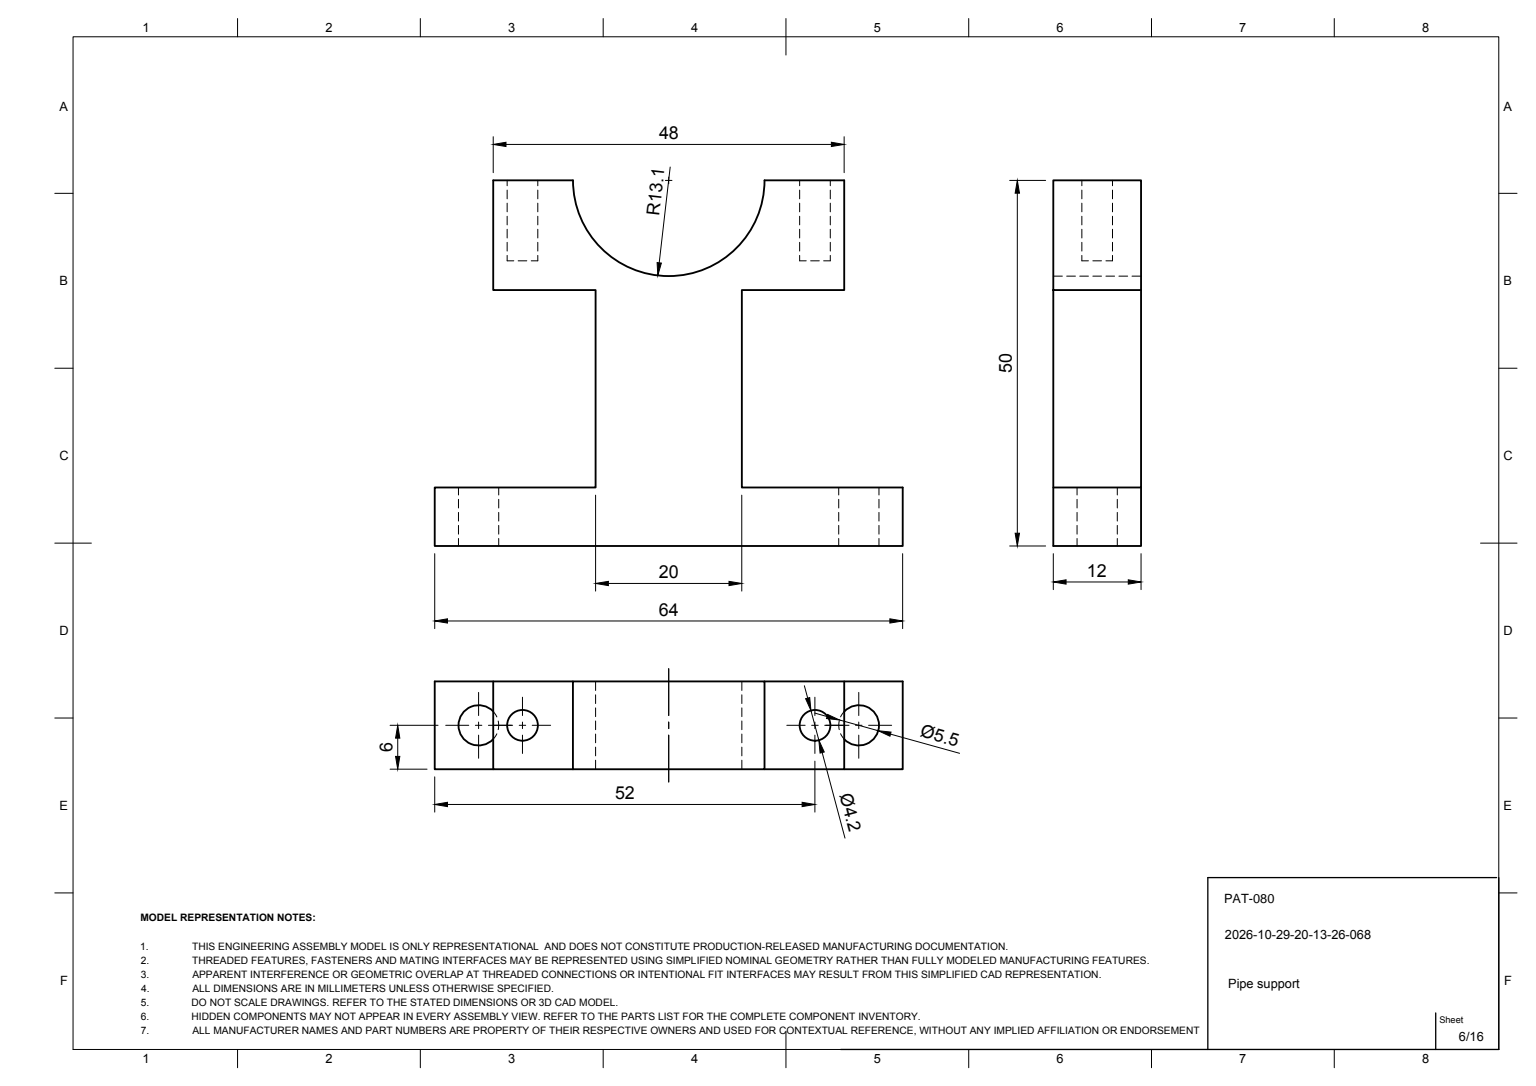
ISO-10303-21;
HEADER;
/* Generated by software containing ST-Developer
 * from STEP Tools, Inc. (www.steptools.com) 
 */

FILE_DESCRIPTION(
/* description */ ('PAT-080'),
/* implementation_level */ '2;1');

FILE_NAME(
/* name */ 'Pipe support.step',
/* time_stamp */ '2026-10-29T20:13:47-07:00',
/* author */ (''),
/* organization */ (''),
/* preprocessor_version */ 'ST-DEVELOPER v20.2',
/* originating_system */ 'Autodesk Translation Framework v15.17.0.0',
/* authorisation */ '');

FILE_SCHEMA (('AUTOMOTIVE_DESIGN { 1 0 10303 214 3 1 1 }'));
ENDSEC;

DATA;
#10=MECHANICAL_DESIGN_GEOMETRIC_PRESENTATION_REPRESENTATION('',(#249),#6878);
#211=SHAPE_REPRESENTATION_RELATIONSHIP('SRR','None',#6967,#230);
#230=ADVANCED_BREP_SHAPE_REPRESENTATION('',(#268),#6862);
#249=STYLED_ITEM('',(#7122),#268);
#268=MANIFOLD_SOLID_BREP('Body1',#3865);
#289=FACE_BOUND('',#765,.T.);
#290=FACE_BOUND('',#767,.T.);
#291=FACE_BOUND('',#769,.T.);
#292=FACE_BOUND('',#777,.T.);
#293=FACE_BOUND('',#780,.T.);
#294=FACE_BOUND('',#781,.T.);
#375=PLANE('',#4132);
#376=PLANE('',#4136);
#377=PLANE('',#4146);
#378=PLANE('',#4147);
#379=PLANE('',#4148);
#380=PLANE('',#4149);
#381=PLANE('',#4150);
#382=PLANE('',#4151);
#383=PLANE('',#4152);
#384=PLANE('',#4153);
#385=PLANE('',#4154);
#386=PLANE('',#4155);
#387=PLANE('',#4156);
#388=PLANE('',#4157);
#389=PLANE('',#4158);
#390=PLANE('',#4159);
#391=PLANE('',#4160);
#522=FACE_OUTER_BOUND('',#756,.T.);
#523=FACE_OUTER_BOUND('',#757,.T.);
#524=FACE_OUTER_BOUND('',#758,.T.);
#525=FACE_OUTER_BOUND('',#759,.T.);
#526=FACE_OUTER_BOUND('',#760,.T.);
#527=FACE_OUTER_BOUND('',#761,.T.);
#528=FACE_OUTER_BOUND('',#762,.T.);
#529=FACE_OUTER_BOUND('',#763,.T.);
#530=FACE_OUTER_BOUND('',#764,.T.);
#531=FACE_OUTER_BOUND('',#766,.T.);
#532=FACE_OUTER_BOUND('',#768,.T.);
#533=FACE_OUTER_BOUND('',#770,.T.);
#534=FACE_OUTER_BOUND('',#771,.T.);
#535=FACE_OUTER_BOUND('',#772,.T.);
#536=FACE_OUTER_BOUND('',#773,.T.);
#537=FACE_OUTER_BOUND('',#774,.T.);
#538=FACE_OUTER_BOUND('',#775,.T.);
#539=FACE_OUTER_BOUND('',#776,.T.);
#540=FACE_OUTER_BOUND('',#778,.T.);
#541=FACE_OUTER_BOUND('',#779,.T.);
#542=FACE_OUTER_BOUND('',#782,.T.);
#543=FACE_OUTER_BOUND('',#783,.T.);
#756=EDGE_LOOP('',(#2704,#2705,#2706,#2707));
#757=EDGE_LOOP('',(#2708));
#758=EDGE_LOOP('',(#2709,#2710,#2711,#2712));
#759=EDGE_LOOP('',(#2713));
#760=EDGE_LOOP('',(#2714,#2715,#2716,#2717));
#761=EDGE_LOOP('',(#2718,#2719,#2720,#2721));
#762=EDGE_LOOP('',(#2722,#2723,#2724,#2725));
#763=EDGE_LOOP('',(#2726,#2727,#2728,#2729,#2730,#2731,#2732,#2733,#2734,
#2735,#2736,#2737,#2738,#2739));
#764=EDGE_LOOP('',(#2740,#2741,#2742,#2743));
#765=EDGE_LOOP('',(#2744));
#766=EDGE_LOOP('',(#2745,#2746,#2747,#2748));
#767=EDGE_LOOP('',(#2749));
#768=EDGE_LOOP('',(#2750,#2751,#2752,#2753));
#769=EDGE_LOOP('',(#2754));
#770=EDGE_LOOP('',(#2755,#2756,#2757,#2758));
#771=EDGE_LOOP('',(#2759,#2760,#2761,#2762));
#772=EDGE_LOOP('',(#2763,#2764,#2765,#2766));
#773=EDGE_LOOP('',(#2767,#2768,#2769,#2770));
#774=EDGE_LOOP('',(#2771,#2772,#2773,#2774));
#775=EDGE_LOOP('',(#2775,#2776,#2777,#2778));
#776=EDGE_LOOP('',(#2779,#2780,#2781,#2782));
#777=EDGE_LOOP('',(#2783));
#778=EDGE_LOOP('',(#2784,#2785,#2786,#2787));
#779=EDGE_LOOP('',(#2788,#2789,#2790,#2791));
#780=EDGE_LOOP('',(#2792));
#781=EDGE_LOOP('',(#2793));
#782=EDGE_LOOP('',(#2794,#2795,#2796,#2797));
#783=EDGE_LOOP('',(#2798,#2799,#2800,#2801,#2802,#2803,#2804,#2805,#2806,
#2807,#2808,#2809,#2810,#2811));
#1068=LINE('',#5840,#1383);
#1069=LINE('',#5847,#1384);
#1070=LINE('',#5854,#1385);
#1071=LINE('',#5860,#1386);
#1072=LINE('',#5865,#1387);
#1073=LINE('',#5869,#1388);
#1074=LINE('',#5873,#1389);
#1075=LINE('',#5875,#1390);
#1076=LINE('',#5877,#1391);
#1077=LINE('',#5879,#1392);
#1078=LINE('',#5881,#1393);
#1079=LINE('',#5883,#1394);
#1080=LINE('',#5885,#1395);
#1081=LINE('',#5887,#1396);
#1082=LINE('',#5889,#1397);
#1083=LINE('',#5891,#1398);
#1084=LINE('',#5893,#1399);
#1085=LINE('',#5895,#1400);
#1086=LINE('',#5896,#1401);
#1087=LINE('',#5899,#1402);
#1088=LINE('',#5900,#1403);
#1089=LINE('',#5903,#1404);
#1090=LINE('',#5904,#1405);
#1091=LINE('',#5908,#1406);
#1092=LINE('',#5909,#1407);
#1093=LINE('',#5910,#1408);
#1094=LINE('',#5913,#1409);
#1095=LINE('',#5914,#1410);
#1096=LINE('',#5917,#1411);
#1097=LINE('',#5918,#1412);
#1098=LINE('',#5920,#1413);
#1099=LINE('',#5923,#1414);
#1100=LINE('',#5924,#1415);
#1101=LINE('',#5927,#1416);
#1102=LINE('',#5928,#1417);
#1103=LINE('',#5931,#1418);
#1104=LINE('',#5932,#1419);
#1105=LINE('',#5935,#1420);
#1106=LINE('',#5936,#1421);
#1107=LINE('',#5939,#1422);
#1108=LINE('',#5940,#1423);
#1109=LINE('',#5943,#1424);
#1110=LINE('',#5944,#1425);
#1111=LINE('',#5946,#1426);
#1383=VECTOR('',#4648,0.21);
#1384=VECTOR('',#4657,0.21);
#1385=VECTOR('',#4666,0.275);
#1386=VECTOR('',#4673,0.275);
#1387=VECTOR('',#4678,1.);
#1388=VECTOR('',#4681,1.);
#1389=VECTOR('',#4686,1.);
#1390=VECTOR('',#4687,1.);
#1391=VECTOR('',#4688,1.);
#1392=VECTOR('',#4689,1.);
#1393=VECTOR('',#4690,1.);
#1394=VECTOR('',#4691,1.);
#1395=VECTOR('',#4692,1.);
#1396=VECTOR('',#4693,1.);
#1397=VECTOR('',#4694,1.);
#1398=VECTOR('',#4695,1.);
#1399=VECTOR('',#4696,1.);
#1400=VECTOR('',#4697,1.);
#1401=VECTOR('',#4698,1.);
#1402=VECTOR('',#4701,1.);
#1403=VECTOR('',#4702,1.);
#1404=VECTOR('',#4705,1.);
#1405=VECTOR('',#4706,1.);
#1406=VECTOR('',#4709,1.);
#1407=VECTOR('',#4710,1.);
#1408=VECTOR('',#4711,1.);
#1409=VECTOR('',#4714,1.);
#1410=VECTOR('',#4715,1.);
#1411=VECTOR('',#4718,1.);
#1412=VECTOR('',#4719,1.);
#1413=VECTOR('',#4722,1.);
#1414=VECTOR('',#4725,1.);
#1415=VECTOR('',#4726,1.);
#1416=VECTOR('',#4729,1.);
#1417=VECTOR('',#4730,1.);
#1418=VECTOR('',#4733,1.);
#1419=VECTOR('',#4734,1.);
#1420=VECTOR('',#4737,1.);
#1421=VECTOR('',#4738,1.);
#1422=VECTOR('',#4741,1.);
#1423=VECTOR('',#4742,1.);
#1424=VECTOR('',#4745,1.);
#1425=VECTOR('',#4746,1.);
#1426=VECTOR('',#4749,1.);
#1666=CIRCLE('',#4130,0.21);
#1667=CIRCLE('',#4131,0.21);
#1668=CIRCLE('',#4134,0.21);
#1669=CIRCLE('',#4135,0.21);
#1670=CIRCLE('',#4138,0.275);
#1671=CIRCLE('',#4139,0.275);
#1672=CIRCLE('',#4141,0.275);
#1673=CIRCLE('',#4142,0.275);
#1674=CIRCLE('',#4144,1.31);
#1675=CIRCLE('',#4145,1.31);
#1842=VERTEX_POINT('',#5837);
#1843=VERTEX_POINT('',#5839);
#1844=VERTEX_POINT('',#5844);
#1845=VERTEX_POINT('',#5846);
#1846=VERTEX_POINT('',#5851);
#1847=VERTEX_POINT('',#5853);
#1848=VERTEX_POINT('',#5857);
#1849=VERTEX_POINT('',#5859);
#1850=VERTEX_POINT('',#5863);
#1851=VERTEX_POINT('',#5864);
#1852=VERTEX_POINT('',#5866);
#1853=VERTEX_POINT('',#5868);
#1854=VERTEX_POINT('',#5872);
#1855=VERTEX_POINT('',#5874);
#1856=VERTEX_POINT('',#5876);
#1857=VERTEX_POINT('',#5878);
#1858=VERTEX_POINT('',#5880);
#1859=VERTEX_POINT('',#5882);
#1860=VERTEX_POINT('',#5884);
#1861=VERTEX_POINT('',#5886);
#1862=VERTEX_POINT('',#5888);
#1863=VERTEX_POINT('',#5890);
#1864=VERTEX_POINT('',#5892);
#1865=VERTEX_POINT('',#5894);
#1866=VERTEX_POINT('',#5898);
#1867=VERTEX_POINT('',#5902);
#1868=VERTEX_POINT('',#5906);
#1869=VERTEX_POINT('',#5907);
#1870=VERTEX_POINT('',#5912);
#1871=VERTEX_POINT('',#5916);
#1872=VERTEX_POINT('',#5922);
#1873=VERTEX_POINT('',#5926);
#1874=VERTEX_POINT('',#5930);
#1875=VERTEX_POINT('',#5934);
#1876=VERTEX_POINT('',#5938);
#1877=VERTEX_POINT('',#5942);
#2175=EDGE_CURVE('',#1842,#1842,#1666,.T.);
#2176=EDGE_CURVE('',#1842,#1843,#1068,.T.);
#2177=EDGE_CURVE('',#1843,#1843,#1667,.T.);
#2178=EDGE_CURVE('',#1844,#1844,#1668,.T.);
#2179=EDGE_CURVE('',#1844,#1845,#1069,.T.);
#2180=EDGE_CURVE('',#1845,#1845,#1669,.T.);
#2181=EDGE_CURVE('',#1846,#1846,#1670,.T.);
#2182=EDGE_CURVE('',#1846,#1847,#1070,.T.);
#2183=EDGE_CURVE('',#1847,#1847,#1671,.T.);
#2184=EDGE_CURVE('',#1848,#1848,#1672,.T.);
#2185=EDGE_CURVE('',#1848,#1849,#1071,.T.);
#2186=EDGE_CURVE('',#1849,#1849,#1673,.T.);
#2187=EDGE_CURVE('',#1850,#1851,#1072,.T.);
#2188=EDGE_CURVE('',#1852,#1850,#1674,.T.);
#2189=EDGE_CURVE('',#1853,#1852,#1073,.T.);
#2190=EDGE_CURVE('',#1851,#1853,#1675,.T.);
#2191=EDGE_CURVE('',#1850,#1854,#1074,.T.);
#2192=EDGE_CURVE('',#1854,#1855,#1075,.T.);
#2193=EDGE_CURVE('',#1855,#1856,#1076,.T.);
#2194=EDGE_CURVE('',#1856,#1857,#1077,.T.);
#2195=EDGE_CURVE('',#1857,#1858,#1078,.T.);
#2196=EDGE_CURVE('',#1858,#1859,#1079,.T.);
#2197=EDGE_CURVE('',#1859,#1860,#1080,.T.);
#2198=EDGE_CURVE('',#1860,#1861,#1081,.T.);
#2199=EDGE_CURVE('',#1861,#1862,#1082,.T.);
#2200=EDGE_CURVE('',#1862,#1863,#1083,.T.);
#2201=EDGE_CURVE('',#1863,#1864,#1084,.T.);
#2202=EDGE_CURVE('',#1864,#1865,#1085,.T.);
#2203=EDGE_CURVE('',#1865,#1852,#1086,.T.);
#2204=EDGE_CURVE('',#1851,#1866,#1087,.T.);
#2205=EDGE_CURVE('',#1866,#1854,#1088,.T.);
#2206=EDGE_CURVE('',#1867,#1865,#1089,.T.);
#2207=EDGE_CURVE('',#1867,#1853,#1090,.T.);
#2208=EDGE_CURVE('',#1868,#1869,#1091,.T.);
#2209=EDGE_CURVE('',#1869,#1858,#1092,.T.);
#2210=EDGE_CURVE('',#1868,#1857,#1093,.T.);
#2211=EDGE_CURVE('',#1870,#1868,#1094,.T.);
#2212=EDGE_CURVE('',#1870,#1856,#1095,.T.);
#2213=EDGE_CURVE('',#1871,#1870,#1096,.T.);
#2214=EDGE_CURVE('',#1871,#1855,#1097,.T.);
#2215=EDGE_CURVE('',#1866,#1871,#1098,.T.);
#2216=EDGE_CURVE('',#1872,#1867,#1099,.T.);
#2217=EDGE_CURVE('',#1872,#1864,#1100,.T.);
#2218=EDGE_CURVE('',#1873,#1872,#1101,.T.);
#2219=EDGE_CURVE('',#1873,#1863,#1102,.T.);
#2220=EDGE_CURVE('',#1874,#1873,#1103,.T.);
#2221=EDGE_CURVE('',#1874,#1862,#1104,.T.);
#2222=EDGE_CURVE('',#1875,#1874,#1105,.T.);
#2223=EDGE_CURVE('',#1875,#1861,#1106,.T.);
#2224=EDGE_CURVE('',#1876,#1875,#1107,.T.);
#2225=EDGE_CURVE('',#1876,#1860,#1108,.T.);
#2226=EDGE_CURVE('',#1877,#1876,#1109,.T.);
#2227=EDGE_CURVE('',#1877,#1859,#1110,.T.);
#2228=EDGE_CURVE('',#1869,#1877,#1111,.T.);
#2704=ORIENTED_EDGE('',*,*,#2175,.F.);
#2705=ORIENTED_EDGE('',*,*,#2176,.T.);
#2706=ORIENTED_EDGE('',*,*,#2177,.F.);
#2707=ORIENTED_EDGE('',*,*,#2176,.F.);
#2708=ORIENTED_EDGE('',*,*,#2175,.T.);
#2709=ORIENTED_EDGE('',*,*,#2178,.F.);
#2710=ORIENTED_EDGE('',*,*,#2179,.T.);
#2711=ORIENTED_EDGE('',*,*,#2180,.F.);
#2712=ORIENTED_EDGE('',*,*,#2179,.F.);
#2713=ORIENTED_EDGE('',*,*,#2178,.T.);
#2714=ORIENTED_EDGE('',*,*,#2181,.F.);
#2715=ORIENTED_EDGE('',*,*,#2182,.T.);
#2716=ORIENTED_EDGE('',*,*,#2183,.F.);
#2717=ORIENTED_EDGE('',*,*,#2182,.F.);
#2718=ORIENTED_EDGE('',*,*,#2184,.F.);
#2719=ORIENTED_EDGE('',*,*,#2185,.T.);
#2720=ORIENTED_EDGE('',*,*,#2186,.F.);
#2721=ORIENTED_EDGE('',*,*,#2185,.F.);
#2722=ORIENTED_EDGE('',*,*,#2187,.F.);
#2723=ORIENTED_EDGE('',*,*,#2188,.F.);
#2724=ORIENTED_EDGE('',*,*,#2189,.F.);
#2725=ORIENTED_EDGE('',*,*,#2190,.F.);
#2726=ORIENTED_EDGE('',*,*,#2188,.T.);
#2727=ORIENTED_EDGE('',*,*,#2191,.T.);
#2728=ORIENTED_EDGE('',*,*,#2192,.T.);
#2729=ORIENTED_EDGE('',*,*,#2193,.T.);
#2730=ORIENTED_EDGE('',*,*,#2194,.T.);
#2731=ORIENTED_EDGE('',*,*,#2195,.T.);
#2732=ORIENTED_EDGE('',*,*,#2196,.T.);
#2733=ORIENTED_EDGE('',*,*,#2197,.T.);
#2734=ORIENTED_EDGE('',*,*,#2198,.T.);
#2735=ORIENTED_EDGE('',*,*,#2199,.T.);
#2736=ORIENTED_EDGE('',*,*,#2200,.T.);
#2737=ORIENTED_EDGE('',*,*,#2201,.T.);
#2738=ORIENTED_EDGE('',*,*,#2202,.T.);
#2739=ORIENTED_EDGE('',*,*,#2203,.T.);
#2740=ORIENTED_EDGE('',*,*,#2187,.T.);
#2741=ORIENTED_EDGE('',*,*,#2204,.T.);
#2742=ORIENTED_EDGE('',*,*,#2205,.T.);
#2743=ORIENTED_EDGE('',*,*,#2191,.F.);
#2744=ORIENTED_EDGE('',*,*,#2177,.T.);
#2745=ORIENTED_EDGE('',*,*,#2189,.T.);
#2746=ORIENTED_EDGE('',*,*,#2203,.F.);
#2747=ORIENTED_EDGE('',*,*,#2206,.F.);
#2748=ORIENTED_EDGE('',*,*,#2207,.T.);
#2749=ORIENTED_EDGE('',*,*,#2180,.T.);
#2750=ORIENTED_EDGE('',*,*,#2208,.T.);
#2751=ORIENTED_EDGE('',*,*,#2209,.T.);
#2752=ORIENTED_EDGE('',*,*,#2195,.F.);
#2753=ORIENTED_EDGE('',*,*,#2210,.F.);
#2754=ORIENTED_EDGE('',*,*,#2183,.T.);
#2755=ORIENTED_EDGE('',*,*,#2211,.T.);
#2756=ORIENTED_EDGE('',*,*,#2210,.T.);
#2757=ORIENTED_EDGE('',*,*,#2194,.F.);
#2758=ORIENTED_EDGE('',*,*,#2212,.F.);
#2759=ORIENTED_EDGE('',*,*,#2213,.T.);
#2760=ORIENTED_EDGE('',*,*,#2212,.T.);
#2761=ORIENTED_EDGE('',*,*,#2193,.F.);
#2762=ORIENTED_EDGE('',*,*,#2214,.F.);
#2763=ORIENTED_EDGE('',*,*,#2215,.T.);
#2764=ORIENTED_EDGE('',*,*,#2214,.T.);
#2765=ORIENTED_EDGE('',*,*,#2192,.F.);
#2766=ORIENTED_EDGE('',*,*,#2205,.F.);
#2767=ORIENTED_EDGE('',*,*,#2216,.T.);
#2768=ORIENTED_EDGE('',*,*,#2206,.T.);
#2769=ORIENTED_EDGE('',*,*,#2202,.F.);
#2770=ORIENTED_EDGE('',*,*,#2217,.F.);
#2771=ORIENTED_EDGE('',*,*,#2218,.T.);
#2772=ORIENTED_EDGE('',*,*,#2217,.T.);
#2773=ORIENTED_EDGE('',*,*,#2201,.F.);
#2774=ORIENTED_EDGE('',*,*,#2219,.F.);
#2775=ORIENTED_EDGE('',*,*,#2220,.T.);
#2776=ORIENTED_EDGE('',*,*,#2219,.T.);
#2777=ORIENTED_EDGE('',*,*,#2200,.F.);
#2778=ORIENTED_EDGE('',*,*,#2221,.F.);
#2779=ORIENTED_EDGE('',*,*,#2222,.T.);
#2780=ORIENTED_EDGE('',*,*,#2221,.T.);
#2781=ORIENTED_EDGE('',*,*,#2199,.F.);
#2782=ORIENTED_EDGE('',*,*,#2223,.F.);
#2783=ORIENTED_EDGE('',*,*,#2186,.T.);
#2784=ORIENTED_EDGE('',*,*,#2224,.T.);
#2785=ORIENTED_EDGE('',*,*,#2223,.T.);
#2786=ORIENTED_EDGE('',*,*,#2198,.F.);
#2787=ORIENTED_EDGE('',*,*,#2225,.F.);
#2788=ORIENTED_EDGE('',*,*,#2226,.T.);
#2789=ORIENTED_EDGE('',*,*,#2225,.T.);
#2790=ORIENTED_EDGE('',*,*,#2197,.F.);
#2791=ORIENTED_EDGE('',*,*,#2227,.F.);
#2792=ORIENTED_EDGE('',*,*,#2181,.T.);
#2793=ORIENTED_EDGE('',*,*,#2184,.T.);
#2794=ORIENTED_EDGE('',*,*,#2228,.T.);
#2795=ORIENTED_EDGE('',*,*,#2227,.T.);
#2796=ORIENTED_EDGE('',*,*,#2196,.F.);
#2797=ORIENTED_EDGE('',*,*,#2209,.F.);
#2798=ORIENTED_EDGE('',*,*,#2190,.T.);
#2799=ORIENTED_EDGE('',*,*,#2207,.F.);
#2800=ORIENTED_EDGE('',*,*,#2216,.F.);
#2801=ORIENTED_EDGE('',*,*,#2218,.F.);
#2802=ORIENTED_EDGE('',*,*,#2220,.F.);
#2803=ORIENTED_EDGE('',*,*,#2222,.F.);
#2804=ORIENTED_EDGE('',*,*,#2224,.F.);
#2805=ORIENTED_EDGE('',*,*,#2226,.F.);
#2806=ORIENTED_EDGE('',*,*,#2228,.F.);
#2807=ORIENTED_EDGE('',*,*,#2208,.F.);
#2808=ORIENTED_EDGE('',*,*,#2211,.F.);
#2809=ORIENTED_EDGE('',*,*,#2213,.F.);
#2810=ORIENTED_EDGE('',*,*,#2215,.F.);
#2811=ORIENTED_EDGE('',*,*,#2204,.F.);
#3574=CYLINDRICAL_SURFACE('',#4129,0.21);
#3575=CYLINDRICAL_SURFACE('',#4133,0.21);
#3576=CYLINDRICAL_SURFACE('',#4137,0.275);
#3577=CYLINDRICAL_SURFACE('',#4140,0.275);
#3578=CYLINDRICAL_SURFACE('',#4143,1.31);
#3658=ADVANCED_FACE('',(#522),#3574,.F.);
#3659=ADVANCED_FACE('',(#523),#375,.T.);
#3660=ADVANCED_FACE('',(#524),#3575,.F.);
#3661=ADVANCED_FACE('',(#525),#376,.T.);
#3662=ADVANCED_FACE('',(#526),#3576,.F.);
#3663=ADVANCED_FACE('',(#527),#3577,.F.);
#3664=ADVANCED_FACE('',(#528),#3578,.F.);
#3665=ADVANCED_FACE('',(#529),#377,.T.);
#3666=ADVANCED_FACE('',(#530,#289),#378,.T.);
#3667=ADVANCED_FACE('',(#531,#290),#379,.T.);
#3668=ADVANCED_FACE('',(#532,#291),#380,.T.);
#3669=ADVANCED_FACE('',(#533),#381,.T.);
#3670=ADVANCED_FACE('',(#534),#382,.T.);
#3671=ADVANCED_FACE('',(#535),#383,.T.);
#3672=ADVANCED_FACE('',(#536),#384,.T.);
#3673=ADVANCED_FACE('',(#537),#385,.T.);
#3674=ADVANCED_FACE('',(#538),#386,.T.);
#3675=ADVANCED_FACE('',(#539,#292),#387,.T.);
#3676=ADVANCED_FACE('',(#540),#388,.T.);
#3677=ADVANCED_FACE('',(#541,#293,#294),#389,.T.);
#3678=ADVANCED_FACE('',(#542),#390,.T.);
#3679=ADVANCED_FACE('',(#543),#391,.F.);
#3865=CLOSED_SHELL('',(#3658,#3659,#3660,#3661,#3662,#3663,#3664,#3665,
#3666,#3667,#3668,#3669,#3670,#3671,#3672,#3673,#3674,#3675,#3676,#3677,
#3678,#3679));
#4128=AXIS2_PLACEMENT_3D('',#5835,#4642,#4643);
#4129=AXIS2_PLACEMENT_3D('',#5836,#4644,#4645);
#4130=AXIS2_PLACEMENT_3D('',#5838,#4646,#4647);
#4131=AXIS2_PLACEMENT_3D('',#5841,#4649,#4650);
#4132=AXIS2_PLACEMENT_3D('',#5842,#4651,#4652);
#4133=AXIS2_PLACEMENT_3D('',#5843,#4653,#4654);
#4134=AXIS2_PLACEMENT_3D('',#5845,#4655,#4656);
#4135=AXIS2_PLACEMENT_3D('',#5848,#4658,#4659);
#4136=AXIS2_PLACEMENT_3D('',#5849,#4660,#4661);
#4137=AXIS2_PLACEMENT_3D('',#5850,#4662,#4663);
#4138=AXIS2_PLACEMENT_3D('',#5852,#4664,#4665);
#4139=AXIS2_PLACEMENT_3D('',#5855,#4667,#4668);
#4140=AXIS2_PLACEMENT_3D('',#5856,#4669,#4670);
#4141=AXIS2_PLACEMENT_3D('',#5858,#4671,#4672);
#4142=AXIS2_PLACEMENT_3D('',#5861,#4674,#4675);
#4143=AXIS2_PLACEMENT_3D('',#5862,#4676,#4677);
#4144=AXIS2_PLACEMENT_3D('',#5867,#4679,#4680);
#4145=AXIS2_PLACEMENT_3D('',#5870,#4682,#4683);
#4146=AXIS2_PLACEMENT_3D('',#5871,#4684,#4685);
#4147=AXIS2_PLACEMENT_3D('',#5897,#4699,#4700);
#4148=AXIS2_PLACEMENT_3D('',#5901,#4703,#4704);
#4149=AXIS2_PLACEMENT_3D('',#5905,#4707,#4708);
#4150=AXIS2_PLACEMENT_3D('',#5911,#4712,#4713);
#4151=AXIS2_PLACEMENT_3D('',#5915,#4716,#4717);
#4152=AXIS2_PLACEMENT_3D('',#5919,#4720,#4721);
#4153=AXIS2_PLACEMENT_3D('',#5921,#4723,#4724);
#4154=AXIS2_PLACEMENT_3D('',#5925,#4727,#4728);
#4155=AXIS2_PLACEMENT_3D('',#5929,#4731,#4732);
#4156=AXIS2_PLACEMENT_3D('',#5933,#4735,#4736);
#4157=AXIS2_PLACEMENT_3D('',#5937,#4739,#4740);
#4158=AXIS2_PLACEMENT_3D('',#5941,#4743,#4744);
#4159=AXIS2_PLACEMENT_3D('',#5945,#4747,#4748);
#4160=AXIS2_PLACEMENT_3D('',#5947,#4750,#4751);
#4642=DIRECTION('axis',(0.,0.,1.));
#4643=DIRECTION('refdir',(1.,0.,0.));
#4644=DIRECTION('center_axis',(0.,0.,1.));
#4645=DIRECTION('ref_axis',(1.,0.,0.));
#4646=DIRECTION('center_axis',(0.,0.,1.));
#4647=DIRECTION('ref_axis',(1.,0.,0.));
#4648=DIRECTION('',(0.,0.,1.));
#4649=DIRECTION('center_axis',(0.,0.,-1.));
#4650=DIRECTION('ref_axis',(1.,0.,0.));
#4651=DIRECTION('center_axis',(0.,0.,1.));
#4652=DIRECTION('ref_axis',(1.,0.,0.));
#4653=DIRECTION('center_axis',(0.,0.,1.));
#4654=DIRECTION('ref_axis',(1.,0.,0.));
#4655=DIRECTION('center_axis',(0.,0.,1.));
#4656=DIRECTION('ref_axis',(1.,0.,0.));
#4657=DIRECTION('',(0.,0.,1.));
#4658=DIRECTION('center_axis',(0.,0.,-1.));
#4659=DIRECTION('ref_axis',(1.,0.,0.));
#4660=DIRECTION('center_axis',(0.,0.,1.));
#4661=DIRECTION('ref_axis',(1.,0.,0.));
#4662=DIRECTION('center_axis',(0.,0.,1.));
#4663=DIRECTION('ref_axis',(1.,0.,0.));
#4664=DIRECTION('center_axis',(0.,0.,1.));
#4665=DIRECTION('ref_axis',(1.,0.,0.));
#4666=DIRECTION('',(0.,0.,1.));
#4667=DIRECTION('center_axis',(0.,0.,-1.));
#4668=DIRECTION('ref_axis',(1.,0.,0.));
#4669=DIRECTION('center_axis',(0.,0.,1.));
#4670=DIRECTION('ref_axis',(1.,0.,0.));
#4671=DIRECTION('center_axis',(0.,0.,1.));
#4672=DIRECTION('ref_axis',(1.,0.,0.));
#4673=DIRECTION('',(0.,0.,1.));
#4674=DIRECTION('center_axis',(0.,0.,-1.));
#4675=DIRECTION('ref_axis',(1.,0.,0.));
#4676=DIRECTION('center_axis',(1.,0.,0.));
#4677=DIRECTION('ref_axis',(0.,0.,-1.));
#4678=DIRECTION('',(-1.,0.,0.));
#4679=DIRECTION('center_axis',(-1.,0.,0.));
#4680=DIRECTION('ref_axis',(0.,0.,-1.));
#4681=DIRECTION('',(1.,0.,0.));
#4682=DIRECTION('center_axis',(1.,0.,0.));
#4683=DIRECTION('ref_axis',(0.,0.,-1.));
#4684=DIRECTION('center_axis',(1.,0.,0.));
#4685=DIRECTION('ref_axis',(0.,0.,-1.));
#4686=DIRECTION('',(0.,-1.,0.));
#4687=DIRECTION('',(0.,0.,-1.));
#4688=DIRECTION('',(0.,1.,0.));
#4689=DIRECTION('',(0.,0.,-1.));
#4690=DIRECTION('',(0.,-1.,0.));
#4691=DIRECTION('',(0.,0.,-1.));
#4692=DIRECTION('',(0.,1.,0.));
#4693=DIRECTION('',(0.,0.,1.));
#4694=DIRECTION('',(0.,-1.,0.));
#4695=DIRECTION('',(0.,0.,1.));
#4696=DIRECTION('',(0.,1.,0.));
#4697=DIRECTION('',(0.,0.,1.));
#4698=DIRECTION('',(0.,-1.,0.));
#4699=DIRECTION('center_axis',(0.,0.,1.));
#4700=DIRECTION('ref_axis',(0.,-1.,0.));
#4701=DIRECTION('',(0.,-1.,0.));
#4702=DIRECTION('',(1.,0.,0.));
#4703=DIRECTION('center_axis',(0.,0.,1.));
#4704=DIRECTION('ref_axis',(0.,-1.,0.));
#4705=DIRECTION('',(1.,0.,0.));
#4706=DIRECTION('',(0.,-1.,0.));
#4707=DIRECTION('center_axis',(0.,0.,1.));
#4708=DIRECTION('ref_axis',(0.,-1.,0.));
#4709=DIRECTION('',(0.,-1.,0.));
#4710=DIRECTION('',(1.,0.,0.));
#4711=DIRECTION('',(1.,0.,0.));
#4712=DIRECTION('center_axis',(0.,-1.,0.));
#4713=DIRECTION('ref_axis',(0.,0.,-1.));
#4714=DIRECTION('',(0.,0.,-1.));
#4715=DIRECTION('',(1.,0.,0.));
#4716=DIRECTION('center_axis',(0.,0.,-1.));
#4717=DIRECTION('ref_axis',(0.,1.,0.));
#4718=DIRECTION('',(0.,1.,0.));
#4719=DIRECTION('',(1.,0.,0.));
#4720=DIRECTION('center_axis',(0.,-1.,0.));
#4721=DIRECTION('ref_axis',(0.,0.,-1.));
#4722=DIRECTION('',(0.,0.,-1.));
#4723=DIRECTION('center_axis',(0.,1.,0.));
#4724=DIRECTION('ref_axis',(0.,0.,1.));
#4725=DIRECTION('',(0.,0.,1.));
#4726=DIRECTION('',(1.,0.,0.));
#4727=DIRECTION('center_axis',(0.,0.,-1.));
#4728=DIRECTION('ref_axis',(0.,1.,0.));
#4729=DIRECTION('',(0.,1.,0.));
#4730=DIRECTION('',(1.,0.,0.));
#4731=DIRECTION('center_axis',(0.,1.,0.));
#4732=DIRECTION('ref_axis',(0.,0.,1.));
#4733=DIRECTION('',(0.,0.,1.));
#4734=DIRECTION('',(1.,0.,0.));
#4735=DIRECTION('center_axis',(0.,0.,1.));
#4736=DIRECTION('ref_axis',(0.,-1.,0.));
#4737=DIRECTION('',(0.,-1.,0.));
#4738=DIRECTION('',(1.,0.,0.));
#4739=DIRECTION('center_axis',(0.,1.,0.));
#4740=DIRECTION('ref_axis',(0.,0.,1.));
#4741=DIRECTION('',(0.,0.,1.));
#4742=DIRECTION('',(1.,0.,0.));
#4743=DIRECTION('center_axis',(0.,0.,-1.));
#4744=DIRECTION('ref_axis',(0.,1.,0.));
#4745=DIRECTION('',(0.,1.,0.));
#4746=DIRECTION('',(1.,0.,0.));
#4747=DIRECTION('center_axis',(0.,-1.,0.));
#4748=DIRECTION('ref_axis',(0.,0.,-1.));
#4749=DIRECTION('',(0.,0.,-1.));
#4750=DIRECTION('center_axis',(1.,0.,0.));
#4751=DIRECTION('ref_axis',(0.,0.,-1.));
#5835=CARTESIAN_POINT('',(0.,0.,0.));
#5836=CARTESIAN_POINT('Origin',(-4.5,-2.,4.9));
#5837=CARTESIAN_POINT('',(-4.71,-2.,4.9));
#5838=CARTESIAN_POINT('Origin',(-4.5,-2.,4.9));
#5839=CARTESIAN_POINT('',(-4.71,-2.,6.));
#5840=CARTESIAN_POINT('',(-4.71,-2.,4.9));
#5841=CARTESIAN_POINT('Origin',(-4.5,-2.,6.));
#5842=CARTESIAN_POINT('Origin',(-4.5,-2.,4.9));
#5843=CARTESIAN_POINT('Origin',(-4.5,2.,4.9));
#5844=CARTESIAN_POINT('',(-4.71,2.,4.9));
#5845=CARTESIAN_POINT('Origin',(-4.5,2.,4.9));
#5846=CARTESIAN_POINT('',(-4.71,2.,6.));
#5847=CARTESIAN_POINT('',(-4.71,2.,4.9));
#5848=CARTESIAN_POINT('Origin',(-4.5,2.,6.));
#5849=CARTESIAN_POINT('Origin',(-4.5,2.,4.9));
#5850=CARTESIAN_POINT('Origin',(-4.5,-2.6,0.9));
#5851=CARTESIAN_POINT('',(-4.775,-2.6,1.));
#5852=CARTESIAN_POINT('Origin',(-4.5,-2.6,1.));
#5853=CARTESIAN_POINT('',(-4.775,-2.6,1.8));
#5854=CARTESIAN_POINT('',(-4.775,-2.6,0.9));
#5855=CARTESIAN_POINT('Origin',(-4.5,-2.6,1.8));
#5856=CARTESIAN_POINT('Origin',(-4.5,2.6,0.9));
#5857=CARTESIAN_POINT('',(-4.775,2.6,1.));
#5858=CARTESIAN_POINT('Origin',(-4.5,2.6,1.));
#5859=CARTESIAN_POINT('',(-4.775,2.6,1.8));
#5860=CARTESIAN_POINT('',(-4.775,2.6,0.9));
#5861=CARTESIAN_POINT('Origin',(-4.5,2.6,1.8));
#5862=CARTESIAN_POINT('Origin',(-5.2,0.,6.));
#5863=CARTESIAN_POINT('',(-3.9,-1.31,6.));
#5864=CARTESIAN_POINT('',(-5.1,-1.31,6.));
#5865=CARTESIAN_POINT('',(-5.2,-1.31,6.));
#5866=CARTESIAN_POINT('',(-3.9,1.31,6.));
#5867=CARTESIAN_POINT('Origin',(-3.9,0.,6.));
#5868=CARTESIAN_POINT('',(-5.1,1.31,6.));
#5869=CARTESIAN_POINT('',(-5.2,1.31,6.));
#5870=CARTESIAN_POINT('Origin',(-5.1,0.,6.));
#5871=CARTESIAN_POINT('Origin',(-3.9,0.,3.5));
#5872=CARTESIAN_POINT('',(-3.9,-2.4,6.));
#5873=CARTESIAN_POINT('',(-3.9,2.4,6.));
#5874=CARTESIAN_POINT('',(-3.9,-2.4,4.5));
#5875=CARTESIAN_POINT('',(-3.9,-2.4,6.));
#5876=CARTESIAN_POINT('',(-3.9,-1.,4.5));
#5877=CARTESIAN_POINT('',(-3.9,-2.4,4.5));
#5878=CARTESIAN_POINT('',(-3.9,-1.,1.8));
#5879=CARTESIAN_POINT('',(-3.9,-1.,4.5));
#5880=CARTESIAN_POINT('',(-3.9,-3.2,1.8));
#5881=CARTESIAN_POINT('',(-3.9,-1.,1.8));
#5882=CARTESIAN_POINT('',(-3.9,-3.2,1.));
#5883=CARTESIAN_POINT('',(-3.9,-3.2,1.8));
#5884=CARTESIAN_POINT('',(-3.9,3.2,1.));
#5885=CARTESIAN_POINT('',(-3.9,-3.2,1.));
#5886=CARTESIAN_POINT('',(-3.9,3.2,1.8));
#5887=CARTESIAN_POINT('',(-3.9,3.2,1.));
#5888=CARTESIAN_POINT('',(-3.9,1.,1.8));
#5889=CARTESIAN_POINT('',(-3.9,3.2,1.8));
#5890=CARTESIAN_POINT('',(-3.9,1.,4.5));
#5891=CARTESIAN_POINT('',(-3.9,1.,1.8));
#5892=CARTESIAN_POINT('',(-3.9,2.4,4.5));
#5893=CARTESIAN_POINT('',(-3.9,1.,4.5));
#5894=CARTESIAN_POINT('',(-3.9,2.4,6.));
#5895=CARTESIAN_POINT('',(-3.9,2.4,4.5));
#5896=CARTESIAN_POINT('',(-3.9,2.4,6.));
#5897=CARTESIAN_POINT('Origin',(-5.1,2.4,6.));
#5898=CARTESIAN_POINT('',(-5.1,-2.4,6.));
#5899=CARTESIAN_POINT('',(-5.1,2.4,6.));
#5900=CARTESIAN_POINT('',(-5.1,-2.4,6.));
#5901=CARTESIAN_POINT('Origin',(-5.1,2.4,6.));
#5902=CARTESIAN_POINT('',(-5.1,2.4,6.));
#5903=CARTESIAN_POINT('',(-5.1,2.4,6.));
#5904=CARTESIAN_POINT('',(-5.1,2.4,6.));
#5905=CARTESIAN_POINT('Origin',(-5.1,-1.,1.8));
#5906=CARTESIAN_POINT('',(-5.1,-1.,1.8));
#5907=CARTESIAN_POINT('',(-5.1,-3.2,1.8));
#5908=CARTESIAN_POINT('',(-5.1,-1.,1.8));
#5909=CARTESIAN_POINT('',(-5.1,-3.2,1.8));
#5910=CARTESIAN_POINT('',(-5.1,-1.,1.8));
#5911=CARTESIAN_POINT('Origin',(-5.1,-1.,4.5));
#5912=CARTESIAN_POINT('',(-5.1,-1.,4.5));
#5913=CARTESIAN_POINT('',(-5.1,-1.,4.5));
#5914=CARTESIAN_POINT('',(-5.1,-1.,4.5));
#5915=CARTESIAN_POINT('Origin',(-5.1,-2.4,4.5));
#5916=CARTESIAN_POINT('',(-5.1,-2.4,4.5));
#5917=CARTESIAN_POINT('',(-5.1,-2.4,4.5));
#5918=CARTESIAN_POINT('',(-5.1,-2.4,4.5));
#5919=CARTESIAN_POINT('Origin',(-5.1,-2.4,6.));
#5920=CARTESIAN_POINT('',(-5.1,-2.4,6.));
#5921=CARTESIAN_POINT('Origin',(-5.1,2.4,4.5));
#5922=CARTESIAN_POINT('',(-5.1,2.4,4.5));
#5923=CARTESIAN_POINT('',(-5.1,2.4,4.5));
#5924=CARTESIAN_POINT('',(-5.1,2.4,4.5));
#5925=CARTESIAN_POINT('Origin',(-5.1,1.,4.5));
#5926=CARTESIAN_POINT('',(-5.1,1.,4.5));
#5927=CARTESIAN_POINT('',(-5.1,1.,4.5));
#5928=CARTESIAN_POINT('',(-5.1,1.,4.5));
#5929=CARTESIAN_POINT('Origin',(-5.1,1.,1.8));
#5930=CARTESIAN_POINT('',(-5.1,1.,1.8));
#5931=CARTESIAN_POINT('',(-5.1,1.,1.8));
#5932=CARTESIAN_POINT('',(-5.1,1.,1.8));
#5933=CARTESIAN_POINT('Origin',(-5.1,3.2,1.8));
#5934=CARTESIAN_POINT('',(-5.1,3.2,1.8));
#5935=CARTESIAN_POINT('',(-5.1,3.2,1.8));
#5936=CARTESIAN_POINT('',(-5.1,3.2,1.8));
#5937=CARTESIAN_POINT('Origin',(-5.1,3.2,1.));
#5938=CARTESIAN_POINT('',(-5.1,3.2,1.));
#5939=CARTESIAN_POINT('',(-5.1,3.2,1.));
#5940=CARTESIAN_POINT('',(-5.1,3.2,1.));
#5941=CARTESIAN_POINT('Origin',(-5.1,-3.2,1.));
#5942=CARTESIAN_POINT('',(-5.1,-3.2,1.));
#5943=CARTESIAN_POINT('',(-5.1,-3.2,1.));
#5944=CARTESIAN_POINT('',(-5.1,-3.2,1.));
#5945=CARTESIAN_POINT('Origin',(-5.1,-3.2,1.8));
#5946=CARTESIAN_POINT('',(-5.1,-3.2,1.8));
#5947=CARTESIAN_POINT('Origin',(-5.1,0.,3.5));
#6841=UNCERTAINTY_MEASURE_WITH_UNIT(LENGTH_MEASURE(0.001),#6879,
'DISTANCE_ACCURACY_VALUE',
'Maximum model space distance between geometric entities at asserted c
onnectivities');
#6857=UNCERTAINTY_MEASURE_WITH_UNIT(LENGTH_MEASURE(0.001),#6879,
'DISTANCE_ACCURACY_VALUE',
'Maximum model space distance between geometric entities at asserted c
onnectivities');
#6862=(
GEOMETRIC_REPRESENTATION_CONTEXT(3)
GLOBAL_UNCERTAINTY_ASSIGNED_CONTEXT((#6841))
GLOBAL_UNIT_ASSIGNED_CONTEXT((#6879,#6881,#6882))
REPRESENTATION_CONTEXT('','3D')
);
#6878=(
GEOMETRIC_REPRESENTATION_CONTEXT(3)
GLOBAL_UNCERTAINTY_ASSIGNED_CONTEXT((#6857))
GLOBAL_UNIT_ASSIGNED_CONTEXT((#6879,#6881,#6882))
REPRESENTATION_CONTEXT('','3D')
);
#6879=(
LENGTH_UNIT()
NAMED_UNIT(*)
SI_UNIT(.CENTI.,.METRE.)
);
#6881=(
NAMED_UNIT(*)
PLANE_ANGLE_UNIT()
SI_UNIT($,.RADIAN.)
);
#6882=(
NAMED_UNIT(*)
SI_UNIT($,.STERADIAN.)
SOLID_ANGLE_UNIT()
);
#6887=SHAPE_DEFINITION_REPRESENTATION(#6907,#6967);
#6907=PRODUCT_DEFINITION_SHAPE('',$,#6988);
#6967=SHAPE_REPRESENTATION('',(#4128),#6862);
#6983=PRODUCT_DEFINITION_CONTEXT('part definition',#7045,'design');
#6988=PRODUCT_DEFINITION('Pipe support','Pipe support',#7008,
#6983);
#7008=PRODUCT_DEFINITION_FORMATION('',$,#7051);
#7045=APPLICATION_CONTEXT(
'Core Data for Automotive Mechanical Design Process');
#7046=PRODUCT_CONTEXT('part definition',#7045,'mechanical');
#7051=PRODUCT('Pipe support','Pipe support','Pipe support',
(#7046));
#7116=COLOUR_RGB('Sky Blue',0.24,0.69,0.87);
#7117=FILL_AREA_STYLE_COLOUR('',#7116);
#7118=FILL_AREA_STYLE('',(#7117));
#7119=SURFACE_STYLE_FILL_AREA(#7118);
#7120=SURFACE_SIDE_STYLE('',(#7119));
#7121=SURFACE_STYLE_USAGE(.BOTH.,#7120);
#7122=PRESENTATION_STYLE_ASSIGNMENT((#7121));
ENDSEC;
END-ISO-10303-21;
